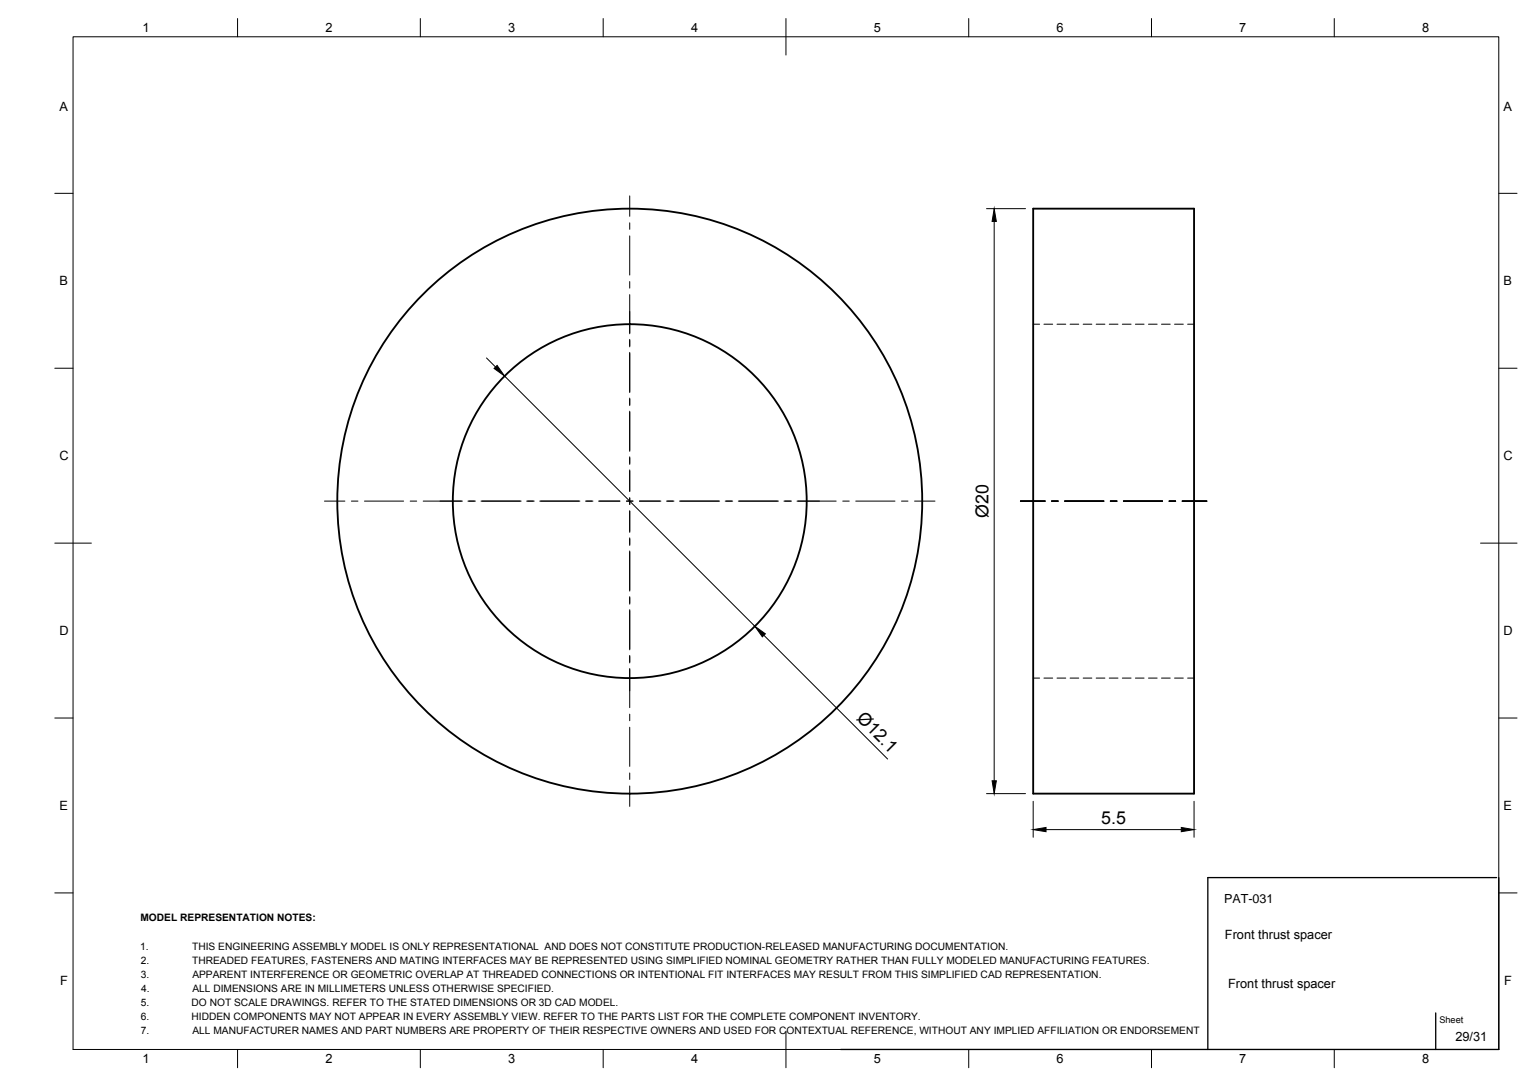
ISO-10303-21;
HEADER;
/* Generated by software containing ST-Developer
 * from STEP Tools, Inc. (www.steptools.com) 
 */

FILE_DESCRIPTION(
/* description */ ('Double-row support with tensioned shaft'),
/* implementation_level */ '2;1');

FILE_NAME(
/* name */ 'Front thrust spacer.step',
/* time_stamp */ '2026-10-27T10:50:35-07:00',
/* author */ (''),
/* organization */ (''),
/* preprocessor_version */ 'ST-DEVELOPER v20.2',
/* originating_system */ 'Autodesk Translation Framework v15.17.0.0',
/* authorisation */ '');

FILE_SCHEMA (('AUTOMOTIVE_DESIGN { 1 0 10303 214 3 1 1 }'));
ENDSEC;

DATA;
#10=MECHANICAL_DESIGN_GEOMETRIC_PRESENTATION_REPRESENTATION('',(#506),#11559);
#441=SHAPE_REPRESENTATION_RELATIONSHIP('SRR','None',#11751,#473);
#473=ADVANCED_BREP_SHAPE_REPRESENTATION('',(#536),#11553);
#506=STYLED_ITEM('',(#11960),#536);
#536=MANIFOLD_SOLID_BREP('Body1',#6354);
#658=FACE_BOUND('',#1662,.T.);
#659=FACE_BOUND('',#1664,.T.);
#871=PLANE('',#7269);
#872=PLANE('',#7270);
#1199=FACE_OUTER_BOUND('',#1659,.T.);
#1200=FACE_OUTER_BOUND('',#1660,.T.);
#1201=FACE_OUTER_BOUND('',#1661,.T.);
#1202=FACE_OUTER_BOUND('',#1663,.T.);
#1659=EDGE_LOOP('',(#5610,#5611,#5612,#5613));
#1660=EDGE_LOOP('',(#5614,#5615,#5616,#5617));
#1661=EDGE_LOOP('',(#5618));
#1662=EDGE_LOOP('',(#5619));
#1663=EDGE_LOOP('',(#5620));
#1664=EDGE_LOOP('',(#5621));
#2184=LINE('',#11128,#2731);
#2185=LINE('',#11134,#2732);
#2731=VECTOR('',#8917,0.605);
#2732=VECTOR('',#8924,1.);
#2996=CIRCLE('',#7264,0.605);
#2997=CIRCLE('',#7265,0.605);
#2998=CIRCLE('',#7267,1.);
#2999=CIRCLE('',#7268,1.);
#3457=VERTEX_POINT('',#11125);
#3458=VERTEX_POINT('',#11127);
#3459=VERTEX_POINT('',#11131);
#3460=VERTEX_POINT('',#11133);
#4190=EDGE_CURVE('',#3457,#3457,#2996,.T.);
#4191=EDGE_CURVE('',#3457,#3458,#2184,.T.);
#4192=EDGE_CURVE('',#3458,#3458,#2997,.T.);
#4193=EDGE_CURVE('',#3459,#3459,#2998,.T.);
#4194=EDGE_CURVE('',#3459,#3460,#2185,.T.);
#4195=EDGE_CURVE('',#3460,#3460,#2999,.T.);
#5610=ORIENTED_EDGE('',*,*,#4190,.F.);
#5611=ORIENTED_EDGE('',*,*,#4191,.T.);
#5612=ORIENTED_EDGE('',*,*,#4192,.T.);
#5613=ORIENTED_EDGE('',*,*,#4191,.F.);
#5614=ORIENTED_EDGE('',*,*,#4193,.F.);
#5615=ORIENTED_EDGE('',*,*,#4194,.T.);
#5616=ORIENTED_EDGE('',*,*,#4195,.T.);
#5617=ORIENTED_EDGE('',*,*,#4194,.F.);
#5618=ORIENTED_EDGE('',*,*,#4193,.T.);
#5619=ORIENTED_EDGE('',*,*,#4190,.T.);
#5620=ORIENTED_EDGE('',*,*,#4195,.F.);
#5621=ORIENTED_EDGE('',*,*,#4192,.F.);
#5966=CYLINDRICAL_SURFACE('',#7263,0.605);
#5967=CYLINDRICAL_SURFACE('',#7266,1.);
#6262=ADVANCED_FACE('',(#1199),#5966,.F.);
#6263=ADVANCED_FACE('',(#1200),#5967,.T.);
#6264=ADVANCED_FACE('',(#1201,#658),#871,.T.);
#6265=ADVANCED_FACE('',(#1202,#659),#872,.F.);
#6354=CLOSED_SHELL('',(#6262,#6263,#6264,#6265));
#7262=AXIS2_PLACEMENT_3D('',#11123,#8911,#8912);
#7263=AXIS2_PLACEMENT_3D('',#11124,#8913,#8914);
#7264=AXIS2_PLACEMENT_3D('',#11126,#8915,#8916);
#7265=AXIS2_PLACEMENT_3D('',#11129,#8918,#8919);
#7266=AXIS2_PLACEMENT_3D('',#11130,#8920,#8921);
#7267=AXIS2_PLACEMENT_3D('',#11132,#8922,#8923);
#7268=AXIS2_PLACEMENT_3D('',#11135,#8925,#8926);
#7269=AXIS2_PLACEMENT_3D('',#11136,#8927,#8928);
#7270=AXIS2_PLACEMENT_3D('',#11137,#8929,#8930);
#8911=DIRECTION('axis',(0.,0.,1.));
#8912=DIRECTION('refdir',(1.,0.,0.));
#8913=DIRECTION('center_axis',(0.,1.,0.));
#8914=DIRECTION('ref_axis',(1.,0.,0.));
#8915=DIRECTION('center_axis',(0.,-1.,0.));
#8916=DIRECTION('ref_axis',(1.,0.,0.));
#8917=DIRECTION('',(0.,-1.,0.));
#8918=DIRECTION('center_axis',(0.,-1.,0.));
#8919=DIRECTION('ref_axis',(1.,0.,0.));
#8920=DIRECTION('center_axis',(0.,1.,0.));
#8921=DIRECTION('ref_axis',(1.,0.,0.));
#8922=DIRECTION('center_axis',(0.,1.,0.));
#8923=DIRECTION('ref_axis',(1.,0.,0.));
#8924=DIRECTION('',(0.,-1.,0.));
#8925=DIRECTION('center_axis',(0.,1.,0.));
#8926=DIRECTION('ref_axis',(1.,0.,0.));
#8927=DIRECTION('center_axis',(0.,1.,0.));
#8928=DIRECTION('ref_axis',(1.,0.,0.));
#8929=DIRECTION('center_axis',(0.,1.,0.));
#8930=DIRECTION('ref_axis',(1.,0.,0.));
#11123=CARTESIAN_POINT('',(0.,0.,0.));
#11124=CARTESIAN_POINT('Origin',(0.,20.45,10.));
#11125=CARTESIAN_POINT('',(-0.605,21.,10.));
#11126=CARTESIAN_POINT('Origin',(0.,21.,10.));
#11127=CARTESIAN_POINT('',(-0.605,20.45,10.));
#11128=CARTESIAN_POINT('',(-0.605,20.45,10.));
#11129=CARTESIAN_POINT('Origin',(0.,20.45,10.));
#11130=CARTESIAN_POINT('Origin',(0.,20.45,10.));
#11131=CARTESIAN_POINT('',(-1.,21.,10.));
#11132=CARTESIAN_POINT('Origin',(0.,21.,10.));
#11133=CARTESIAN_POINT('',(-1.,20.45,10.));
#11134=CARTESIAN_POINT('',(-1.,20.45,10.));
#11135=CARTESIAN_POINT('Origin',(0.,20.45,10.));
#11136=CARTESIAN_POINT('Origin',(0.,21.,10.));
#11137=CARTESIAN_POINT('Origin',(0.,20.45,10.));
#11516=UNCERTAINTY_MEASURE_WITH_UNIT(LENGTH_MEASURE(0.001),#11560,
'DISTANCE_ACCURACY_VALUE',
'Maximum model space distance between geometric entities at asserted c
onnectivities');
#11522=UNCERTAINTY_MEASURE_WITH_UNIT(LENGTH_MEASURE(0.001),#11560,
'DISTANCE_ACCURACY_VALUE',
'Maximum model space distance between geometric entities at asserted c
onnectivities');
#11553=(
GEOMETRIC_REPRESENTATION_CONTEXT(3)
GLOBAL_UNCERTAINTY_ASSIGNED_CONTEXT((#11516))
GLOBAL_UNIT_ASSIGNED_CONTEXT((#11560,#11562,#11563))
REPRESENTATION_CONTEXT('','3D')
);
#11559=(
GEOMETRIC_REPRESENTATION_CONTEXT(3)
GLOBAL_UNCERTAINTY_ASSIGNED_CONTEXT((#11522))
GLOBAL_UNIT_ASSIGNED_CONTEXT((#11560,#11562,#11563))
REPRESENTATION_CONTEXT('','3D')
);
#11560=(
LENGTH_UNIT()
NAMED_UNIT(*)
SI_UNIT(.CENTI.,.METRE.)
);
#11562=(
NAMED_UNIT(*)
PLANE_ANGLE_UNIT()
SI_UNIT($,.RADIAN.)
);
#11563=(
NAMED_UNIT(*)
SI_UNIT($,.STERADIAN.)
SOLID_ANGLE_UNIT()
);
#11594=SHAPE_DEFINITION_REPRESENTATION(#11705,#11751);
#11705=PRODUCT_DEFINITION_SHAPE('',$,#11788);
#11751=SHAPE_REPRESENTATION('',(#7262),#11553);
#11757=PRODUCT_DEFINITION_CONTEXT('part definition',#11867,'design');
#11788=PRODUCT_DEFINITION('Front thrust spacer','Front thrust spacer',#11824,
#11757);
#11824=PRODUCT_DEFINITION_FORMATION('',$,#11899);
#11867=APPLICATION_CONTEXT(
'Core Data for Automotive Mechanical Design Process');
#11868=PRODUCT_CONTEXT('part definition',#11867,'mechanical');
#11899=PRODUCT('Front thrust spacer','Front thrust spacer',
'Front thrust spacer',(#11868));
#11954=COLOUR_RGB('Sky Blue',0.24,0.69,0.87);
#11955=FILL_AREA_STYLE_COLOUR('',#11954);
#11956=FILL_AREA_STYLE('',(#11955));
#11957=SURFACE_STYLE_FILL_AREA(#11956);
#11958=SURFACE_SIDE_STYLE('',(#11957));
#11959=SURFACE_STYLE_USAGE(.BOTH.,#11958);
#11960=PRESENTATION_STYLE_ASSIGNMENT((#11959));
ENDSEC;
END-ISO-10303-21;
